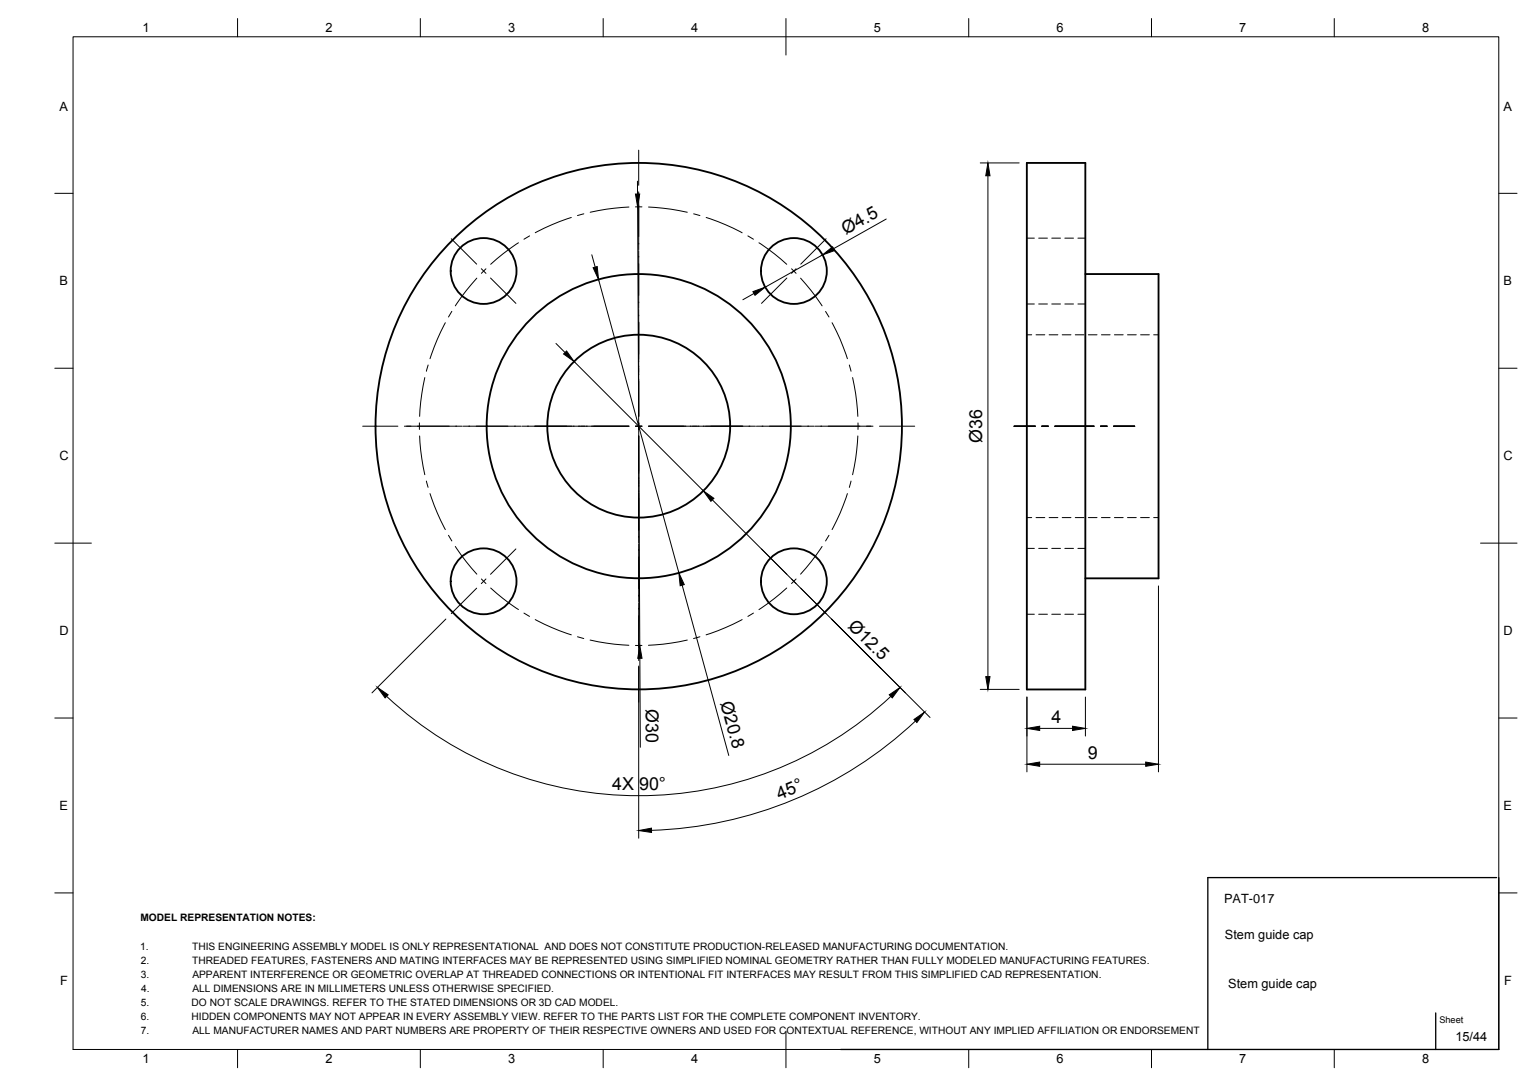
ISO-10303-21;
HEADER;
/* Generated by software containing ST-Developer
 * from STEP Tools, Inc. (www.steptools.com) 
 */

FILE_DESCRIPTION(
/* description */ ('Cam-and-follower valve demonstrator'),
/* implementation_level */ '2;1');

FILE_NAME(
/* name */ 'Stem guide cap.step',
/* time_stamp */ '2026-10-28T03:25:17-07:00',
/* author */ (''),
/* organization */ (''),
/* preprocessor_version */ 'ST-DEVELOPER v20.2',
/* originating_system */ 'Autodesk Translation Framework v15.17.0.0',
/* authorisation */ '');

FILE_SCHEMA (('AUTOMOTIVE_DESIGN { 1 0 10303 214 3 1 1 }'));
ENDSEC;

DATA;
#10=MECHANICAL_DESIGN_GEOMETRIC_PRESENTATION_REPRESENTATION('',(#422),#12896);
#350=SHAPE_REPRESENTATION_RELATIONSHIP('SRR','None',#13066,#386);
#386=ADVANCED_BREP_SHAPE_REPRESENTATION('',(#465),#12866);
#422=STYLED_ITEM('',(#13344),#465);
#465=MANIFOLD_SOLID_BREP('Body1',#6189);
#593=FACE_BOUND('',#1701,.T.);
#594=FACE_BOUND('',#1705,.T.);
#595=FACE_BOUND('',#1706,.T.);
#596=FACE_BOUND('',#1707,.T.);
#597=FACE_BOUND('',#1708,.T.);
#598=FACE_BOUND('',#1709,.T.);
#599=FACE_BOUND('',#1711,.T.);
#600=FACE_BOUND('',#1712,.T.);
#601=FACE_BOUND('',#1713,.T.);
#602=FACE_BOUND('',#1714,.T.);
#603=FACE_BOUND('',#1715,.T.);
#775=CIRCLE('',#6886,0.225);
#776=CIRCLE('',#6887,0.225);
#777=CIRCLE('',#6889,0.225);
#778=CIRCLE('',#6890,0.225);
#779=CIRCLE('',#6892,0.225);
#780=CIRCLE('',#6893,0.225);
#781=CIRCLE('',#6895,0.225);
#782=CIRCLE('',#6896,0.225);
#783=CIRCLE('',#6898,1.04);
#784=CIRCLE('',#6899,1.04);
#785=CIRCLE('',#6901,0.625);
#786=CIRCLE('',#6903,0.625);
#787=CIRCLE('',#6905,1.8);
#788=CIRCLE('',#6906,1.8);
#1031=CYLINDRICAL_SURFACE('',#6885,0.225);
#1032=CYLINDRICAL_SURFACE('',#6888,0.225);
#1033=CYLINDRICAL_SURFACE('',#6891,0.225);
#1034=CYLINDRICAL_SURFACE('',#6894,0.225);
#1035=CYLINDRICAL_SURFACE('',#6897,1.04);
#1036=CYLINDRICAL_SURFACE('',#6902,0.625);
#1037=CYLINDRICAL_SURFACE('',#6904,1.8);
#1229=FACE_OUTER_BOUND('',#1695,.T.);
#1230=FACE_OUTER_BOUND('',#1696,.T.);
#1231=FACE_OUTER_BOUND('',#1697,.T.);
#1232=FACE_OUTER_BOUND('',#1698,.T.);
#1233=FACE_OUTER_BOUND('',#1699,.T.);
#1234=FACE_OUTER_BOUND('',#1700,.T.);
#1235=FACE_OUTER_BOUND('',#1702,.T.);
#1236=FACE_OUTER_BOUND('',#1703,.T.);
#1237=FACE_OUTER_BOUND('',#1704,.T.);
#1238=FACE_OUTER_BOUND('',#1710,.T.);
#1695=EDGE_LOOP('',(#4707,#4708,#4709,#4710));
#1696=EDGE_LOOP('',(#4711,#4712,#4713,#4714));
#1697=EDGE_LOOP('',(#4715,#4716,#4717,#4718));
#1698=EDGE_LOOP('',(#4719,#4720,#4721,#4722));
#1699=EDGE_LOOP('',(#4723,#4724,#4725,#4726));
#1700=EDGE_LOOP('',(#4727));
#1701=EDGE_LOOP('',(#4728));
#1702=EDGE_LOOP('',(#4729,#4730,#4731,#4732));
#1703=EDGE_LOOP('',(#4733,#4734,#4735,#4736));
#1704=EDGE_LOOP('',(#4737));
#1705=EDGE_LOOP('',(#4738));
#1706=EDGE_LOOP('',(#4739));
#1707=EDGE_LOOP('',(#4740));
#1708=EDGE_LOOP('',(#4741));
#1709=EDGE_LOOP('',(#4742));
#1710=EDGE_LOOP('',(#4743));
#1711=EDGE_LOOP('',(#4744));
#1712=EDGE_LOOP('',(#4745));
#1713=EDGE_LOOP('',(#4746));
#1714=EDGE_LOOP('',(#4747));
#1715=EDGE_LOOP('',(#4748));
#2185=LINE('',#10081,#2607);
#2186=LINE('',#10087,#2608);
#2187=LINE('',#10093,#2609);
#2188=LINE('',#10099,#2610);
#2189=LINE('',#10105,#2611);
#2190=LINE('',#10113,#2612);
#2191=LINE('',#10118,#2613);
#2607=VECTOR('',#8134,0.225);
#2608=VECTOR('',#8141,0.225);
#2609=VECTOR('',#8148,0.225);
#2610=VECTOR('',#8155,0.225);
#2611=VECTOR('',#8162,1.04);
#2612=VECTOR('',#8173,0.625);
#2613=VECTOR('',#8178,1.8);
#3043=VERTEX_POINT('',#10078);
#3044=VERTEX_POINT('',#10080);
#3045=VERTEX_POINT('',#10084);
#3046=VERTEX_POINT('',#10086);
#3047=VERTEX_POINT('',#10090);
#3048=VERTEX_POINT('',#10092);
#3049=VERTEX_POINT('',#10096);
#3050=VERTEX_POINT('',#10098);
#3051=VERTEX_POINT('',#10102);
#3052=VERTEX_POINT('',#10104);
#3053=VERTEX_POINT('',#10108);
#3054=VERTEX_POINT('',#10111);
#3055=VERTEX_POINT('',#10115);
#3056=VERTEX_POINT('',#10117);
#3650=EDGE_CURVE('',#3043,#3043,#775,.T.);
#3651=EDGE_CURVE('',#3043,#3044,#2185,.T.);
#3652=EDGE_CURVE('',#3044,#3044,#776,.T.);
#3653=EDGE_CURVE('',#3045,#3045,#777,.T.);
#3654=EDGE_CURVE('',#3045,#3046,#2186,.T.);
#3655=EDGE_CURVE('',#3046,#3046,#778,.T.);
#3656=EDGE_CURVE('',#3047,#3047,#779,.T.);
#3657=EDGE_CURVE('',#3047,#3048,#2187,.T.);
#3658=EDGE_CURVE('',#3048,#3048,#780,.T.);
#3659=EDGE_CURVE('',#3049,#3049,#781,.T.);
#3660=EDGE_CURVE('',#3049,#3050,#2188,.T.);
#3661=EDGE_CURVE('',#3050,#3050,#782,.T.);
#3662=EDGE_CURVE('',#3051,#3051,#783,.T.);
#3663=EDGE_CURVE('',#3051,#3052,#2189,.T.);
#3664=EDGE_CURVE('',#3052,#3052,#784,.T.);
#3665=EDGE_CURVE('',#3053,#3053,#785,.T.);
#3666=EDGE_CURVE('',#3054,#3054,#786,.T.);
#3667=EDGE_CURVE('',#3054,#3053,#2190,.T.);
#3668=EDGE_CURVE('',#3055,#3055,#787,.T.);
#3669=EDGE_CURVE('',#3055,#3056,#2191,.T.);
#3670=EDGE_CURVE('',#3056,#3056,#788,.T.);
#4707=ORIENTED_EDGE('',*,*,#3650,.F.);
#4708=ORIENTED_EDGE('',*,*,#3651,.T.);
#4709=ORIENTED_EDGE('',*,*,#3652,.F.);
#4710=ORIENTED_EDGE('',*,*,#3651,.F.);
#4711=ORIENTED_EDGE('',*,*,#3653,.F.);
#4712=ORIENTED_EDGE('',*,*,#3654,.T.);
#4713=ORIENTED_EDGE('',*,*,#3655,.F.);
#4714=ORIENTED_EDGE('',*,*,#3654,.F.);
#4715=ORIENTED_EDGE('',*,*,#3656,.F.);
#4716=ORIENTED_EDGE('',*,*,#3657,.T.);
#4717=ORIENTED_EDGE('',*,*,#3658,.F.);
#4718=ORIENTED_EDGE('',*,*,#3657,.F.);
#4719=ORIENTED_EDGE('',*,*,#3659,.F.);
#4720=ORIENTED_EDGE('',*,*,#3660,.T.);
#4721=ORIENTED_EDGE('',*,*,#3661,.F.);
#4722=ORIENTED_EDGE('',*,*,#3660,.F.);
#4723=ORIENTED_EDGE('',*,*,#3662,.F.);
#4724=ORIENTED_EDGE('',*,*,#3663,.T.);
#4725=ORIENTED_EDGE('',*,*,#3664,.T.);
#4726=ORIENTED_EDGE('',*,*,#3663,.F.);
#4727=ORIENTED_EDGE('',*,*,#3664,.F.);
#4728=ORIENTED_EDGE('',*,*,#3665,.F.);
#4729=ORIENTED_EDGE('',*,*,#3666,.F.);
#4730=ORIENTED_EDGE('',*,*,#3667,.T.);
#4731=ORIENTED_EDGE('',*,*,#3665,.T.);
#4732=ORIENTED_EDGE('',*,*,#3667,.F.);
#4733=ORIENTED_EDGE('',*,*,#3668,.F.);
#4734=ORIENTED_EDGE('',*,*,#3669,.T.);
#4735=ORIENTED_EDGE('',*,*,#3670,.T.);
#4736=ORIENTED_EDGE('',*,*,#3669,.F.);
#4737=ORIENTED_EDGE('',*,*,#3668,.T.);
#4738=ORIENTED_EDGE('',*,*,#3666,.T.);
#4739=ORIENTED_EDGE('',*,*,#3661,.T.);
#4740=ORIENTED_EDGE('',*,*,#3658,.T.);
#4741=ORIENTED_EDGE('',*,*,#3655,.T.);
#4742=ORIENTED_EDGE('',*,*,#3652,.T.);
#4743=ORIENTED_EDGE('',*,*,#3670,.F.);
#4744=ORIENTED_EDGE('',*,*,#3662,.T.);
#4745=ORIENTED_EDGE('',*,*,#3659,.T.);
#4746=ORIENTED_EDGE('',*,*,#3656,.T.);
#4747=ORIENTED_EDGE('',*,*,#3653,.T.);
#4748=ORIENTED_EDGE('',*,*,#3650,.T.);
#5673=PLANE('',#6900);
#5674=PLANE('',#6907);
#5675=PLANE('',#6908);
#5945=ADVANCED_FACE('',(#1229),#1031,.F.);
#5946=ADVANCED_FACE('',(#1230),#1032,.F.);
#5947=ADVANCED_FACE('',(#1231),#1033,.F.);
#5948=ADVANCED_FACE('',(#1232),#1034,.F.);
#5949=ADVANCED_FACE('',(#1233),#1035,.T.);
#5950=ADVANCED_FACE('',(#1234,#593),#5673,.F.);
#5951=ADVANCED_FACE('',(#1235),#1036,.F.);
#5952=ADVANCED_FACE('',(#1236),#1037,.T.);
#5953=ADVANCED_FACE('',(#1237,#594,#595,#596,#597,#598),#5674,.T.);
#5954=ADVANCED_FACE('',(#1238,#599,#600,#601,#602,#603),#5675,.F.);
#6189=CLOSED_SHELL('',(#5945,#5946,#5947,#5948,#5949,#5950,#5951,#5952,
#5953,#5954));
#6884=AXIS2_PLACEMENT_3D('',#10076,#8128,#8129);
#6885=AXIS2_PLACEMENT_3D('',#10077,#8130,#8131);
#6886=AXIS2_PLACEMENT_3D('',#10079,#8132,#8133);
#6887=AXIS2_PLACEMENT_3D('',#10082,#8135,#8136);
#6888=AXIS2_PLACEMENT_3D('',#10083,#8137,#8138);
#6889=AXIS2_PLACEMENT_3D('',#10085,#8139,#8140);
#6890=AXIS2_PLACEMENT_3D('',#10088,#8142,#8143);
#6891=AXIS2_PLACEMENT_3D('',#10089,#8144,#8145);
#6892=AXIS2_PLACEMENT_3D('',#10091,#8146,#8147);
#6893=AXIS2_PLACEMENT_3D('',#10094,#8149,#8150);
#6894=AXIS2_PLACEMENT_3D('',#10095,#8151,#8152);
#6895=AXIS2_PLACEMENT_3D('',#10097,#8153,#8154);
#6896=AXIS2_PLACEMENT_3D('',#10100,#8156,#8157);
#6897=AXIS2_PLACEMENT_3D('',#10101,#8158,#8159);
#6898=AXIS2_PLACEMENT_3D('',#10103,#8160,#8161);
#6899=AXIS2_PLACEMENT_3D('',#10106,#8163,#8164);
#6900=AXIS2_PLACEMENT_3D('',#10107,#8165,#8166);
#6901=AXIS2_PLACEMENT_3D('',#10109,#8167,#8168);
#6902=AXIS2_PLACEMENT_3D('',#10110,#8169,#8170);
#6903=AXIS2_PLACEMENT_3D('',#10112,#8171,#8172);
#6904=AXIS2_PLACEMENT_3D('',#10114,#8174,#8175);
#6905=AXIS2_PLACEMENT_3D('',#10116,#8176,#8177);
#6906=AXIS2_PLACEMENT_3D('',#10119,#8179,#8180);
#6907=AXIS2_PLACEMENT_3D('',#10120,#8181,#8182);
#6908=AXIS2_PLACEMENT_3D('',#10121,#8183,#8184);
#8128=DIRECTION('axis',(0.,0.,1.));
#8129=DIRECTION('refdir',(1.,0.,0.));
#8130=DIRECTION('center_axis',(0.,0.,1.));
#8131=DIRECTION('ref_axis',(1.,0.,0.));
#8132=DIRECTION('center_axis',(0.,0.,1.));
#8133=DIRECTION('ref_axis',(1.,0.,0.));
#8134=DIRECTION('',(0.,0.,1.));
#8135=DIRECTION('center_axis',(0.,0.,-1.));
#8136=DIRECTION('ref_axis',(1.,0.,0.));
#8137=DIRECTION('center_axis',(0.,0.,1.));
#8138=DIRECTION('ref_axis',(1.,0.,0.));
#8139=DIRECTION('center_axis',(0.,0.,1.));
#8140=DIRECTION('ref_axis',(1.,0.,0.));
#8141=DIRECTION('',(0.,0.,1.));
#8142=DIRECTION('center_axis',(0.,0.,-1.));
#8143=DIRECTION('ref_axis',(1.,0.,0.));
#8144=DIRECTION('center_axis',(0.,0.,1.));
#8145=DIRECTION('ref_axis',(1.,0.,0.));
#8146=DIRECTION('center_axis',(0.,0.,1.));
#8147=DIRECTION('ref_axis',(1.,0.,0.));
#8148=DIRECTION('',(0.,0.,1.));
#8149=DIRECTION('center_axis',(0.,0.,-1.));
#8150=DIRECTION('ref_axis',(1.,0.,0.));
#8151=DIRECTION('center_axis',(0.,0.,1.));
#8152=DIRECTION('ref_axis',(1.,0.,0.));
#8153=DIRECTION('center_axis',(0.,0.,1.));
#8154=DIRECTION('ref_axis',(1.,0.,0.));
#8155=DIRECTION('',(0.,0.,1.));
#8156=DIRECTION('center_axis',(0.,0.,-1.));
#8157=DIRECTION('ref_axis',(1.,0.,0.));
#8158=DIRECTION('center_axis',(0.,0.,1.));
#8159=DIRECTION('ref_axis',(1.,0.,0.));
#8160=DIRECTION('center_axis',(0.,0.,1.));
#8161=DIRECTION('ref_axis',(1.,0.,0.));
#8162=DIRECTION('',(0.,0.,-1.));
#8163=DIRECTION('center_axis',(0.,0.,1.));
#8164=DIRECTION('ref_axis',(1.,0.,0.));
#8165=DIRECTION('center_axis',(0.,0.,1.));
#8166=DIRECTION('ref_axis',(1.,0.,0.));
#8167=DIRECTION('center_axis',(0.,0.,-1.));
#8168=DIRECTION('ref_axis',(1.,0.,0.));
#8169=DIRECTION('center_axis',(0.,0.,1.));
#8170=DIRECTION('ref_axis',(1.,0.,0.));
#8171=DIRECTION('center_axis',(0.,0.,-1.));
#8172=DIRECTION('ref_axis',(1.,0.,0.));
#8173=DIRECTION('',(0.,0.,-1.));
#8174=DIRECTION('center_axis',(0.,0.,1.));
#8175=DIRECTION('ref_axis',(1.,0.,0.));
#8176=DIRECTION('center_axis',(0.,0.,1.));
#8177=DIRECTION('ref_axis',(1.,0.,0.));
#8178=DIRECTION('',(0.,0.,-1.));
#8179=DIRECTION('center_axis',(0.,0.,1.));
#8180=DIRECTION('ref_axis',(1.,0.,0.));
#8181=DIRECTION('center_axis',(0.,0.,1.));
#8182=DIRECTION('ref_axis',(1.,0.,0.));
#8183=DIRECTION('center_axis',(0.,0.,1.));
#8184=DIRECTION('ref_axis',(1.,0.,0.));
#10076=CARTESIAN_POINT('',(0.,0.,0.));
#10077=CARTESIAN_POINT('Origin',(-1.06066017177982,-1.06066017177982,13.9));
#10078=CARTESIAN_POINT('',(-1.28566017177982,-1.06066017177982,14.));
#10079=CARTESIAN_POINT('Origin',(-1.06066017177982,-1.06066017177982,14.));
#10080=CARTESIAN_POINT('',(-1.28566017177982,-1.06066017177982,14.4));
#10081=CARTESIAN_POINT('',(-1.28566017177982,-1.06066017177982,13.9));
#10082=CARTESIAN_POINT('Origin',(-1.06066017177982,-1.06066017177982,14.4));
#10083=CARTESIAN_POINT('Origin',(-1.06066017177982,1.06066017177982,13.9));
#10084=CARTESIAN_POINT('',(-1.28566017177982,1.06066017177982,14.));
#10085=CARTESIAN_POINT('Origin',(-1.06066017177982,1.06066017177982,14.));
#10086=CARTESIAN_POINT('',(-1.28566017177982,1.06066017177982,14.4));
#10087=CARTESIAN_POINT('',(-1.28566017177982,1.06066017177982,13.9));
#10088=CARTESIAN_POINT('Origin',(-1.06066017177982,1.06066017177982,14.4));
#10089=CARTESIAN_POINT('Origin',(1.06066017177982,1.06066017177982,13.9));
#10090=CARTESIAN_POINT('',(0.835660171779821,1.06066017177982,14.));
#10091=CARTESIAN_POINT('Origin',(1.06066017177982,1.06066017177982,14.));
#10092=CARTESIAN_POINT('',(0.835660171779821,1.06066017177982,14.4));
#10093=CARTESIAN_POINT('',(0.835660171779821,1.06066017177982,13.9));
#10094=CARTESIAN_POINT('Origin',(1.06066017177982,1.06066017177982,14.4));
#10095=CARTESIAN_POINT('Origin',(1.06066017177982,-1.06066017177982,13.9));
#10096=CARTESIAN_POINT('',(0.835660171779821,-1.06066017177982,14.));
#10097=CARTESIAN_POINT('Origin',(1.06066017177982,-1.06066017177982,14.));
#10098=CARTESIAN_POINT('',(0.835660171779821,-1.06066017177982,14.4));
#10099=CARTESIAN_POINT('',(0.835660171779821,-1.06066017177982,13.9));
#10100=CARTESIAN_POINT('Origin',(1.06066017177982,-1.06066017177982,14.4));
#10101=CARTESIAN_POINT('Origin',(0.,0.,13.5));
#10102=CARTESIAN_POINT('',(-1.04,-1.27363267111325E-16,14.));
#10103=CARTESIAN_POINT('Origin',(0.,0.,14.));
#10104=CARTESIAN_POINT('',(-1.04,-1.27363267111325E-16,13.5));
#10105=CARTESIAN_POINT('',(-1.04,-1.27363267111325E-16,13.5));
#10106=CARTESIAN_POINT('Origin',(0.,0.,13.5));
#10107=CARTESIAN_POINT('Origin',(0.,0.,13.5));
#10108=CARTESIAN_POINT('',(-0.625,-7.65404249467096E-17,13.5));
#10109=CARTESIAN_POINT('Origin',(0.,0.,13.5));
#10110=CARTESIAN_POINT('Origin',(0.,0.,14.));
#10111=CARTESIAN_POINT('',(-0.625,-7.65404249467096E-17,14.4));
#10112=CARTESIAN_POINT('Origin',(0.,0.,14.4));
#10113=CARTESIAN_POINT('',(-0.625,-7.65404249467096E-17,14.));
#10114=CARTESIAN_POINT('Origin',(0.,0.,14.));
#10115=CARTESIAN_POINT('',(-1.8,-2.20436423846524E-16,14.4));
#10116=CARTESIAN_POINT('Origin',(0.,0.,14.4));
#10117=CARTESIAN_POINT('',(-1.8,-2.20436423846524E-16,14.));
#10118=CARTESIAN_POINT('',(-1.8,-2.20436423846524E-16,14.));
#10119=CARTESIAN_POINT('Origin',(0.,0.,14.));
#10120=CARTESIAN_POINT('Origin',(0.,0.,14.4));
#10121=CARTESIAN_POINT('Origin',(0.,0.,14.));
#12823=UNCERTAINTY_MEASURE_WITH_UNIT(LENGTH_MEASURE(0.001),#12897,
'DISTANCE_ACCURACY_VALUE',
'Maximum model space distance between geometric entities at asserted c
onnectivities');
#12853=UNCERTAINTY_MEASURE_WITH_UNIT(LENGTH_MEASURE(0.001),#12897,
'DISTANCE_ACCURACY_VALUE',
'Maximum model space distance between geometric entities at asserted c
onnectivities');
#12866=(
GEOMETRIC_REPRESENTATION_CONTEXT(3)
GLOBAL_UNCERTAINTY_ASSIGNED_CONTEXT((#12823))
GLOBAL_UNIT_ASSIGNED_CONTEXT((#12897,#12899,#12900))
REPRESENTATION_CONTEXT('','3D')
);
#12896=(
GEOMETRIC_REPRESENTATION_CONTEXT(3)
GLOBAL_UNCERTAINTY_ASSIGNED_CONTEXT((#12853))
GLOBAL_UNIT_ASSIGNED_CONTEXT((#12897,#12899,#12900))
REPRESENTATION_CONTEXT('','3D')
);
#12897=(
LENGTH_UNIT()
NAMED_UNIT(*)
SI_UNIT(.CENTI.,.METRE.)
);
#12899=(
NAMED_UNIT(*)
PLANE_ANGLE_UNIT()
SI_UNIT($,.RADIAN.)
);
#12900=(
NAMED_UNIT(*)
SI_UNIT($,.STERADIAN.)
SOLID_ANGLE_UNIT()
);
#12913=SHAPE_DEFINITION_REPRESENTATION(#12955,#13066);
#12955=PRODUCT_DEFINITION_SHAPE('',$,#13109);
#13066=SHAPE_REPRESENTATION('',(#6884),#12866);
#13096=PRODUCT_DEFINITION_CONTEXT('part definition',#13224,'design');
#13109=PRODUCT_DEFINITION('Stem guide cap','Stem guide cap',#13151,#13096);
#13151=PRODUCT_DEFINITION_FORMATION('',$,#13238);
#13224=APPLICATION_CONTEXT(
'Core Data for Automotive Mechanical Design Process');
#13225=PRODUCT_CONTEXT('part definition',#13224,'mechanical');
#13238=PRODUCT('Stem guide cap','Stem guide cap','Stem guide cap',(#13225));
#13338=COLOUR_RGB('Off White',0.89,0.88,0.83);
#13339=FILL_AREA_STYLE_COLOUR('',#13338);
#13340=FILL_AREA_STYLE('',(#13339));
#13341=SURFACE_STYLE_FILL_AREA(#13340);
#13342=SURFACE_SIDE_STYLE('',(#13341));
#13343=SURFACE_STYLE_USAGE(.BOTH.,#13342);
#13344=PRESENTATION_STYLE_ASSIGNMENT((#13343));
ENDSEC;
END-ISO-10303-21;
